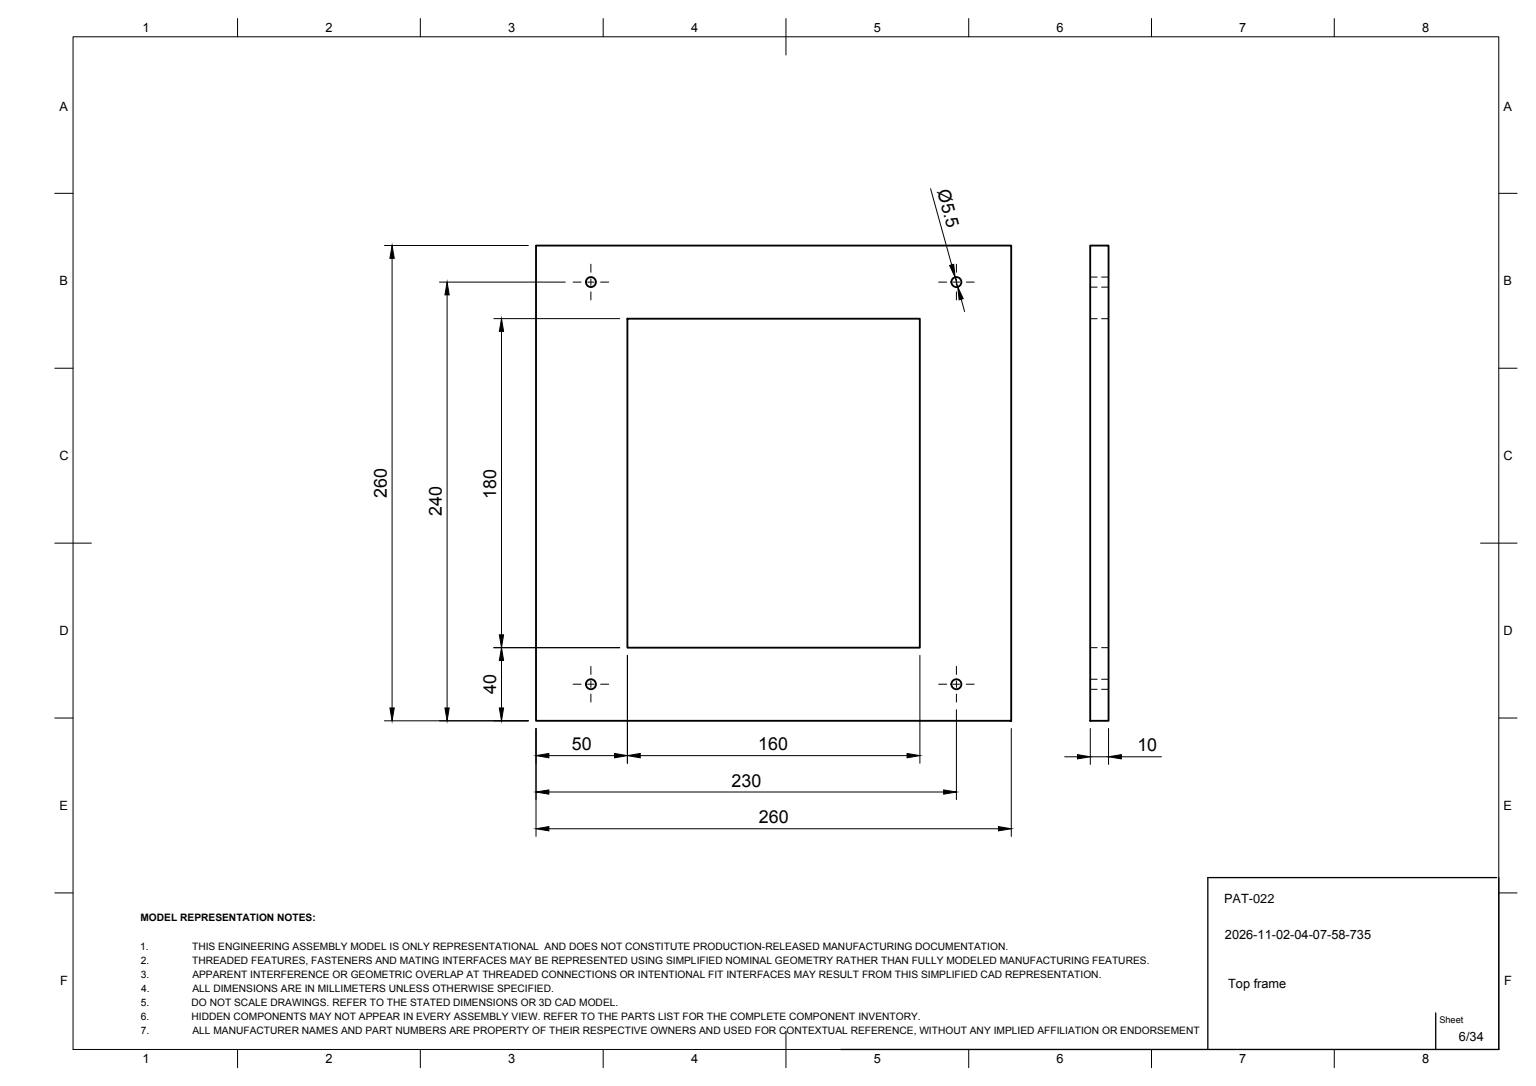
ISO-10303-21;
HEADER;
/* Generated by software containing ST-Developer
 * from STEP Tools, Inc. (www.steptools.com) 
 */

FILE_DESCRIPTION(
/* description */ ('Chute with adjustable gate'),
/* implementation_level */ '2;1');

FILE_NAME(
/* name */ 'Top frame.step',
/* time_stamp */ '2026-10-27T10:52:28-07:00',
/* author */ (''),
/* organization */ (''),
/* preprocessor_version */ 'ST-DEVELOPER v20.2',
/* originating_system */ 'Autodesk Translation Framework v15.17.0.0',
/* authorisation */ '');

FILE_SCHEMA (('AUTOMOTIVE_DESIGN { 1 0 10303 214 3 1 1 }'));
ENDSEC;

DATA;
#10=MECHANICAL_DESIGN_GEOMETRIC_PRESENTATION_REPRESENTATION('',(#415),#13094);
#351=SHAPE_REPRESENTATION_RELATIONSHIP('SRR','None',#13252,#383);
#383=ADVANCED_BREP_SHAPE_REPRESENTATION('',(#447),#13061);
#415=STYLED_ITEM('',(#13474),#447);
#447=MANIFOLD_SOLID_BREP('Body1',#7598);
#482=FACE_BOUND('',#1360,.T.);
#483=FACE_BOUND('',#1361,.T.);
#484=FACE_BOUND('',#1362,.T.);
#485=FACE_BOUND('',#1363,.T.);
#486=FACE_BOUND('',#1364,.T.);
#487=FACE_BOUND('',#1366,.T.);
#488=FACE_BOUND('',#1367,.T.);
#489=FACE_BOUND('',#1368,.T.);
#490=FACE_BOUND('',#1369,.T.);
#491=FACE_BOUND('',#1370,.T.);
#596=PLANE('',#8020);
#597=PLANE('',#8021);
#598=PLANE('',#8022);
#599=PLANE('',#8023);
#600=PLANE('',#8024);
#601=PLANE('',#8025);
#602=PLANE('',#8026);
#603=PLANE('',#8027);
#604=PLANE('',#8028);
#605=PLANE('',#8029);
#924=FACE_OUTER_BOUND('',#1347,.T.);
#925=FACE_OUTER_BOUND('',#1348,.T.);
#926=FACE_OUTER_BOUND('',#1349,.T.);
#927=FACE_OUTER_BOUND('',#1350,.T.);
#928=FACE_OUTER_BOUND('',#1351,.T.);
#929=FACE_OUTER_BOUND('',#1352,.T.);
#930=FACE_OUTER_BOUND('',#1353,.T.);
#931=FACE_OUTER_BOUND('',#1354,.T.);
#932=FACE_OUTER_BOUND('',#1355,.T.);
#933=FACE_OUTER_BOUND('',#1356,.T.);
#934=FACE_OUTER_BOUND('',#1357,.T.);
#935=FACE_OUTER_BOUND('',#1358,.T.);
#936=FACE_OUTER_BOUND('',#1359,.T.);
#937=FACE_OUTER_BOUND('',#1365,.T.);
#1347=EDGE_LOOP('',(#5234,#5235,#5236,#5237));
#1348=EDGE_LOOP('',(#5238,#5239,#5240,#5241));
#1349=EDGE_LOOP('',(#5242,#5243,#5244,#5245));
#1350=EDGE_LOOP('',(#5246,#5247,#5248,#5249));
#1351=EDGE_LOOP('',(#5250,#5251,#5252,#5253));
#1352=EDGE_LOOP('',(#5254,#5255,#5256,#5257));
#1353=EDGE_LOOP('',(#5258,#5259,#5260,#5261));
#1354=EDGE_LOOP('',(#5262,#5263,#5264,#5265));
#1355=EDGE_LOOP('',(#5266,#5267,#5268,#5269));
#1356=EDGE_LOOP('',(#5270,#5271,#5272,#5273));
#1357=EDGE_LOOP('',(#5274,#5275,#5276,#5277));
#1358=EDGE_LOOP('',(#5278,#5279,#5280,#5281));
#1359=EDGE_LOOP('',(#5282,#5283,#5284,#5285));
#1360=EDGE_LOOP('',(#5286,#5287,#5288,#5289));
#1361=EDGE_LOOP('',(#5290));
#1362=EDGE_LOOP('',(#5291));
#1363=EDGE_LOOP('',(#5292));
#1364=EDGE_LOOP('',(#5293));
#1365=EDGE_LOOP('',(#5294,#5295,#5296,#5297));
#1366=EDGE_LOOP('',(#5298,#5299,#5300,#5301));
#1367=EDGE_LOOP('',(#5302));
#1368=EDGE_LOOP('',(#5303));
#1369=EDGE_LOOP('',(#5304));
#1370=EDGE_LOOP('',(#5305));
#1876=LINE('',#10957,#2653);
#1877=LINE('',#10963,#2654);
#1878=LINE('',#10969,#2655);
#1879=LINE('',#10975,#2656);
#1880=LINE('',#10980,#2657);
#1881=LINE('',#10982,#2658);
#1882=LINE('',#10984,#2659);
#1883=LINE('',#10985,#2660);
#1884=LINE('',#10988,#2661);
#1885=LINE('',#10990,#2662);
#1886=LINE('',#10991,#2663);
#1887=LINE('',#10994,#2664);
#1888=LINE('',#10996,#2665);
#1889=LINE('',#10997,#2666);
#1890=LINE('',#10999,#2667);
#1891=LINE('',#11000,#2668);
#1892=LINE('',#11004,#2669);
#1893=LINE('',#11006,#2670);
#1894=LINE('',#11008,#2671);
#1895=LINE('',#11009,#2672);
#1896=LINE('',#11012,#2673);
#1897=LINE('',#11014,#2674);
#1898=LINE('',#11015,#2675);
#1899=LINE('',#11018,#2676);
#1900=LINE('',#11020,#2677);
#1901=LINE('',#11021,#2678);
#1902=LINE('',#11023,#2679);
#1903=LINE('',#11024,#2680);
#2653=VECTOR('',#8762,0.274999999999999);
#2654=VECTOR('',#8769,0.275);
#2655=VECTOR('',#8776,0.275);
#2656=VECTOR('',#8783,0.274999999999999);
#2657=VECTOR('',#8788,1.);
#2658=VECTOR('',#8789,1.);
#2659=VECTOR('',#8790,1.);
#2660=VECTOR('',#8791,1.);
#2661=VECTOR('',#8794,1.);
#2662=VECTOR('',#8795,1.);
#2663=VECTOR('',#8796,1.);
#2664=VECTOR('',#8799,1.);
#2665=VECTOR('',#8800,1.);
#2666=VECTOR('',#8801,1.);
#2667=VECTOR('',#8804,1.);
#2668=VECTOR('',#8805,1.);
#2669=VECTOR('',#8808,1.);
#2670=VECTOR('',#8809,1.);
#2671=VECTOR('',#8810,1.);
#2672=VECTOR('',#8811,1.);
#2673=VECTOR('',#8814,1.);
#2674=VECTOR('',#8815,1.);
#2675=VECTOR('',#8816,1.);
#2676=VECTOR('',#8819,1.);
#2677=VECTOR('',#8820,1.);
#2678=VECTOR('',#8821,1.);
#2679=VECTOR('',#8824,1.);
#2680=VECTOR('',#8825,1.);
#3422=CIRCLE('',#8009,0.274999999999999);
#3423=CIRCLE('',#8010,0.274999999999999);
#3424=CIRCLE('',#8012,0.275);
#3425=CIRCLE('',#8013,0.275);
#3426=CIRCLE('',#8015,0.275);
#3427=CIRCLE('',#8016,0.275);
#3428=CIRCLE('',#8018,0.274999999999999);
#3429=CIRCLE('',#8019,0.274999999999999);
#3609=VERTEX_POINT('',#10954);
#3610=VERTEX_POINT('',#10956);
#3611=VERTEX_POINT('',#10960);
#3612=VERTEX_POINT('',#10962);
#3613=VERTEX_POINT('',#10966);
#3614=VERTEX_POINT('',#10968);
#3615=VERTEX_POINT('',#10972);
#3616=VERTEX_POINT('',#10974);
#3617=VERTEX_POINT('',#10978);
#3618=VERTEX_POINT('',#10979);
#3619=VERTEX_POINT('',#10981);
#3620=VERTEX_POINT('',#10983);
#3621=VERTEX_POINT('',#10987);
#3622=VERTEX_POINT('',#10989);
#3623=VERTEX_POINT('',#10993);
#3624=VERTEX_POINT('',#10995);
#3625=VERTEX_POINT('',#11002);
#3626=VERTEX_POINT('',#11003);
#3627=VERTEX_POINT('',#11005);
#3628=VERTEX_POINT('',#11007);
#3629=VERTEX_POINT('',#11011);
#3630=VERTEX_POINT('',#11013);
#3631=VERTEX_POINT('',#11017);
#3632=VERTEX_POINT('',#11019);
#4250=EDGE_CURVE('',#3609,#3609,#3422,.T.);
#4251=EDGE_CURVE('',#3609,#3610,#1876,.T.);
#4252=EDGE_CURVE('',#3610,#3610,#3423,.T.);
#4253=EDGE_CURVE('',#3611,#3611,#3424,.T.);
#4254=EDGE_CURVE('',#3611,#3612,#1877,.T.);
#4255=EDGE_CURVE('',#3612,#3612,#3425,.T.);
#4256=EDGE_CURVE('',#3613,#3613,#3426,.T.);
#4257=EDGE_CURVE('',#3613,#3614,#1878,.T.);
#4258=EDGE_CURVE('',#3614,#3614,#3427,.T.);
#4259=EDGE_CURVE('',#3615,#3615,#3428,.T.);
#4260=EDGE_CURVE('',#3615,#3616,#1879,.T.);
#4261=EDGE_CURVE('',#3616,#3616,#3429,.T.);
#4262=EDGE_CURVE('',#3617,#3618,#1880,.T.);
#4263=EDGE_CURVE('',#3619,#3617,#1881,.T.);
#4264=EDGE_CURVE('',#3620,#3619,#1882,.T.);
#4265=EDGE_CURVE('',#3620,#3618,#1883,.T.);
#4266=EDGE_CURVE('',#3618,#3621,#1884,.T.);
#4267=EDGE_CURVE('',#3622,#3620,#1885,.T.);
#4268=EDGE_CURVE('',#3622,#3621,#1886,.T.);
#4269=EDGE_CURVE('',#3621,#3623,#1887,.T.);
#4270=EDGE_CURVE('',#3624,#3622,#1888,.T.);
#4271=EDGE_CURVE('',#3624,#3623,#1889,.T.);
#4272=EDGE_CURVE('',#3623,#3617,#1890,.T.);
#4273=EDGE_CURVE('',#3619,#3624,#1891,.T.);
#4274=EDGE_CURVE('',#3625,#3626,#1892,.T.);
#4275=EDGE_CURVE('',#3626,#3627,#1893,.T.);
#4276=EDGE_CURVE('',#3628,#3627,#1894,.T.);
#4277=EDGE_CURVE('',#3625,#3628,#1895,.T.);
#4278=EDGE_CURVE('',#3629,#3625,#1896,.T.);
#4279=EDGE_CURVE('',#3630,#3628,#1897,.T.);
#4280=EDGE_CURVE('',#3629,#3630,#1898,.T.);
#4281=EDGE_CURVE('',#3631,#3629,#1899,.T.);
#4282=EDGE_CURVE('',#3632,#3630,#1900,.T.);
#4283=EDGE_CURVE('',#3631,#3632,#1901,.T.);
#4284=EDGE_CURVE('',#3626,#3631,#1902,.T.);
#4285=EDGE_CURVE('',#3627,#3632,#1903,.T.);
#5234=ORIENTED_EDGE('',*,*,#4250,.F.);
#5235=ORIENTED_EDGE('',*,*,#4251,.T.);
#5236=ORIENTED_EDGE('',*,*,#4252,.F.);
#5237=ORIENTED_EDGE('',*,*,#4251,.F.);
#5238=ORIENTED_EDGE('',*,*,#4253,.F.);
#5239=ORIENTED_EDGE('',*,*,#4254,.T.);
#5240=ORIENTED_EDGE('',*,*,#4255,.F.);
#5241=ORIENTED_EDGE('',*,*,#4254,.F.);
#5242=ORIENTED_EDGE('',*,*,#4256,.F.);
#5243=ORIENTED_EDGE('',*,*,#4257,.T.);
#5244=ORIENTED_EDGE('',*,*,#4258,.F.);
#5245=ORIENTED_EDGE('',*,*,#4257,.F.);
#5246=ORIENTED_EDGE('',*,*,#4259,.F.);
#5247=ORIENTED_EDGE('',*,*,#4260,.T.);
#5248=ORIENTED_EDGE('',*,*,#4261,.F.);
#5249=ORIENTED_EDGE('',*,*,#4260,.F.);
#5250=ORIENTED_EDGE('',*,*,#4262,.F.);
#5251=ORIENTED_EDGE('',*,*,#4263,.F.);
#5252=ORIENTED_EDGE('',*,*,#4264,.F.);
#5253=ORIENTED_EDGE('',*,*,#4265,.T.);
#5254=ORIENTED_EDGE('',*,*,#4266,.F.);
#5255=ORIENTED_EDGE('',*,*,#4265,.F.);
#5256=ORIENTED_EDGE('',*,*,#4267,.F.);
#5257=ORIENTED_EDGE('',*,*,#4268,.T.);
#5258=ORIENTED_EDGE('',*,*,#4269,.F.);
#5259=ORIENTED_EDGE('',*,*,#4268,.F.);
#5260=ORIENTED_EDGE('',*,*,#4270,.F.);
#5261=ORIENTED_EDGE('',*,*,#4271,.T.);
#5262=ORIENTED_EDGE('',*,*,#4272,.F.);
#5263=ORIENTED_EDGE('',*,*,#4271,.F.);
#5264=ORIENTED_EDGE('',*,*,#4273,.F.);
#5265=ORIENTED_EDGE('',*,*,#4263,.T.);
#5266=ORIENTED_EDGE('',*,*,#4274,.T.);
#5267=ORIENTED_EDGE('',*,*,#4275,.T.);
#5268=ORIENTED_EDGE('',*,*,#4276,.F.);
#5269=ORIENTED_EDGE('',*,*,#4277,.F.);
#5270=ORIENTED_EDGE('',*,*,#4278,.T.);
#5271=ORIENTED_EDGE('',*,*,#4277,.T.);
#5272=ORIENTED_EDGE('',*,*,#4279,.F.);
#5273=ORIENTED_EDGE('',*,*,#4280,.F.);
#5274=ORIENTED_EDGE('',*,*,#4281,.T.);
#5275=ORIENTED_EDGE('',*,*,#4280,.T.);
#5276=ORIENTED_EDGE('',*,*,#4282,.F.);
#5277=ORIENTED_EDGE('',*,*,#4283,.F.);
#5278=ORIENTED_EDGE('',*,*,#4284,.T.);
#5279=ORIENTED_EDGE('',*,*,#4283,.T.);
#5280=ORIENTED_EDGE('',*,*,#4285,.F.);
#5281=ORIENTED_EDGE('',*,*,#4275,.F.);
#5282=ORIENTED_EDGE('',*,*,#4285,.T.);
#5283=ORIENTED_EDGE('',*,*,#4282,.T.);
#5284=ORIENTED_EDGE('',*,*,#4279,.T.);
#5285=ORIENTED_EDGE('',*,*,#4276,.T.);
#5286=ORIENTED_EDGE('',*,*,#4269,.T.);
#5287=ORIENTED_EDGE('',*,*,#4272,.T.);
#5288=ORIENTED_EDGE('',*,*,#4262,.T.);
#5289=ORIENTED_EDGE('',*,*,#4266,.T.);
#5290=ORIENTED_EDGE('',*,*,#4261,.T.);
#5291=ORIENTED_EDGE('',*,*,#4258,.T.);
#5292=ORIENTED_EDGE('',*,*,#4255,.T.);
#5293=ORIENTED_EDGE('',*,*,#4252,.T.);
#5294=ORIENTED_EDGE('',*,*,#4284,.F.);
#5295=ORIENTED_EDGE('',*,*,#4274,.F.);
#5296=ORIENTED_EDGE('',*,*,#4278,.F.);
#5297=ORIENTED_EDGE('',*,*,#4281,.F.);
#5298=ORIENTED_EDGE('',*,*,#4270,.T.);
#5299=ORIENTED_EDGE('',*,*,#4267,.T.);
#5300=ORIENTED_EDGE('',*,*,#4264,.T.);
#5301=ORIENTED_EDGE('',*,*,#4273,.T.);
#5302=ORIENTED_EDGE('',*,*,#4259,.T.);
#5303=ORIENTED_EDGE('',*,*,#4256,.T.);
#5304=ORIENTED_EDGE('',*,*,#4253,.T.);
#5305=ORIENTED_EDGE('',*,*,#4250,.T.);
#7110=CYLINDRICAL_SURFACE('',#8008,0.274999999999999);
#7111=CYLINDRICAL_SURFACE('',#8011,0.275);
#7112=CYLINDRICAL_SURFACE('',#8014,0.275);
#7113=CYLINDRICAL_SURFACE('',#8017,0.274999999999999);
#7192=ADVANCED_FACE('',(#924),#7110,.F.);
#7193=ADVANCED_FACE('',(#925),#7111,.F.);
#7194=ADVANCED_FACE('',(#926),#7112,.F.);
#7195=ADVANCED_FACE('',(#927),#7113,.F.);
#7196=ADVANCED_FACE('',(#928),#596,.F.);
#7197=ADVANCED_FACE('',(#929),#597,.F.);
#7198=ADVANCED_FACE('',(#930),#598,.F.);
#7199=ADVANCED_FACE('',(#931),#599,.F.);
#7200=ADVANCED_FACE('',(#932),#600,.T.);
#7201=ADVANCED_FACE('',(#933),#601,.T.);
#7202=ADVANCED_FACE('',(#934),#602,.T.);
#7203=ADVANCED_FACE('',(#935),#603,.T.);
#7204=ADVANCED_FACE('',(#936,#482,#483,#484,#485,#486),#604,.T.);
#7205=ADVANCED_FACE('',(#937,#487,#488,#489,#490,#491),#605,.F.);
#7598=CLOSED_SHELL('',(#7192,#7193,#7194,#7195,#7196,#7197,#7198,#7199,
#7200,#7201,#7202,#7203,#7204,#7205));
#8007=AXIS2_PLACEMENT_3D('',#10952,#8756,#8757);
#8008=AXIS2_PLACEMENT_3D('',#10953,#8758,#8759);
#8009=AXIS2_PLACEMENT_3D('',#10955,#8760,#8761);
#8010=AXIS2_PLACEMENT_3D('',#10958,#8763,#8764);
#8011=AXIS2_PLACEMENT_3D('',#10959,#8765,#8766);
#8012=AXIS2_PLACEMENT_3D('',#10961,#8767,#8768);
#8013=AXIS2_PLACEMENT_3D('',#10964,#8770,#8771);
#8014=AXIS2_PLACEMENT_3D('',#10965,#8772,#8773);
#8015=AXIS2_PLACEMENT_3D('',#10967,#8774,#8775);
#8016=AXIS2_PLACEMENT_3D('',#10970,#8777,#8778);
#8017=AXIS2_PLACEMENT_3D('',#10971,#8779,#8780);
#8018=AXIS2_PLACEMENT_3D('',#10973,#8781,#8782);
#8019=AXIS2_PLACEMENT_3D('',#10976,#8784,#8785);
#8020=AXIS2_PLACEMENT_3D('',#10977,#8786,#8787);
#8021=AXIS2_PLACEMENT_3D('',#10986,#8792,#8793);
#8022=AXIS2_PLACEMENT_3D('',#10992,#8797,#8798);
#8023=AXIS2_PLACEMENT_3D('',#10998,#8802,#8803);
#8024=AXIS2_PLACEMENT_3D('',#11001,#8806,#8807);
#8025=AXIS2_PLACEMENT_3D('',#11010,#8812,#8813);
#8026=AXIS2_PLACEMENT_3D('',#11016,#8817,#8818);
#8027=AXIS2_PLACEMENT_3D('',#11022,#8822,#8823);
#8028=AXIS2_PLACEMENT_3D('',#11025,#8826,#8827);
#8029=AXIS2_PLACEMENT_3D('',#11026,#8828,#8829);
#8756=DIRECTION('axis',(0.,0.,1.));
#8757=DIRECTION('refdir',(1.,0.,0.));
#8758=DIRECTION('center_axis',(0.,0.,1.));
#8759=DIRECTION('ref_axis',(1.,0.,0.));
#8760=DIRECTION('center_axis',(0.,0.,1.));
#8761=DIRECTION('ref_axis',(1.,0.,0.));
#8762=DIRECTION('',(0.,0.,1.));
#8763=DIRECTION('center_axis',(0.,0.,-1.));
#8764=DIRECTION('ref_axis',(1.,0.,0.));
#8765=DIRECTION('center_axis',(0.,0.,1.));
#8766=DIRECTION('ref_axis',(1.,0.,0.));
#8767=DIRECTION('center_axis',(0.,0.,1.));
#8768=DIRECTION('ref_axis',(1.,0.,0.));
#8769=DIRECTION('',(0.,0.,1.));
#8770=DIRECTION('center_axis',(0.,0.,-1.));
#8771=DIRECTION('ref_axis',(1.,0.,0.));
#8772=DIRECTION('center_axis',(0.,0.,1.));
#8773=DIRECTION('ref_axis',(1.,0.,0.));
#8774=DIRECTION('center_axis',(0.,0.,1.));
#8775=DIRECTION('ref_axis',(1.,0.,0.));
#8776=DIRECTION('',(0.,0.,1.));
#8777=DIRECTION('center_axis',(0.,0.,-1.));
#8778=DIRECTION('ref_axis',(1.,0.,0.));
#8779=DIRECTION('center_axis',(0.,0.,1.));
#8780=DIRECTION('ref_axis',(1.,0.,0.));
#8781=DIRECTION('center_axis',(0.,0.,1.));
#8782=DIRECTION('ref_axis',(1.,0.,0.));
#8783=DIRECTION('',(0.,0.,1.));
#8784=DIRECTION('center_axis',(0.,0.,-1.));
#8785=DIRECTION('ref_axis',(1.,0.,0.));
#8786=DIRECTION('center_axis',(0.,-1.,0.));
#8787=DIRECTION('ref_axis',(1.,0.,0.));
#8788=DIRECTION('',(-1.,0.,0.));
#8789=DIRECTION('',(0.,0.,1.));
#8790=DIRECTION('',(1.,0.,0.));
#8791=DIRECTION('',(0.,0.,1.));
#8792=DIRECTION('center_axis',(-1.,0.,0.));
#8793=DIRECTION('ref_axis',(0.,-1.,0.));
#8794=DIRECTION('',(0.,1.,0.));
#8795=DIRECTION('',(0.,-1.,0.));
#8796=DIRECTION('',(0.,0.,1.));
#8797=DIRECTION('center_axis',(0.,1.,0.));
#8798=DIRECTION('ref_axis',(-1.,0.,0.));
#8799=DIRECTION('',(1.,0.,0.));
#8800=DIRECTION('',(-1.,0.,0.));
#8801=DIRECTION('',(0.,0.,1.));
#8802=DIRECTION('center_axis',(1.,0.,0.));
#8803=DIRECTION('ref_axis',(0.,1.,0.));
#8804=DIRECTION('',(0.,-1.,0.));
#8805=DIRECTION('',(0.,1.,0.));
#8806=DIRECTION('center_axis',(0.,1.,0.));
#8807=DIRECTION('ref_axis',(-1.,0.,0.));
#8808=DIRECTION('',(-1.,0.,0.));
#8809=DIRECTION('',(0.,0.,1.));
#8810=DIRECTION('',(-1.,0.,0.));
#8811=DIRECTION('',(0.,0.,1.));
#8812=DIRECTION('center_axis',(1.,0.,0.));
#8813=DIRECTION('ref_axis',(0.,1.,0.));
#8814=DIRECTION('',(0.,1.,0.));
#8815=DIRECTION('',(0.,1.,0.));
#8816=DIRECTION('',(0.,0.,1.));
#8817=DIRECTION('center_axis',(0.,-1.,0.));
#8818=DIRECTION('ref_axis',(1.,0.,0.));
#8819=DIRECTION('',(1.,0.,0.));
#8820=DIRECTION('',(1.,0.,0.));
#8821=DIRECTION('',(0.,0.,1.));
#8822=DIRECTION('center_axis',(-1.,0.,0.));
#8823=DIRECTION('ref_axis',(0.,-1.,0.));
#8824=DIRECTION('',(0.,-1.,0.));
#8825=DIRECTION('',(0.,-1.,0.));
#8826=DIRECTION('center_axis',(0.,0.,1.));
#8827=DIRECTION('ref_axis',(1.,0.,0.));
#8828=DIRECTION('center_axis',(0.,0.,1.));
#8829=DIRECTION('ref_axis',(1.,0.,0.));
#10952=CARTESIAN_POINT('',(0.,0.,0.));
#10953=CARTESIAN_POINT('Origin',(23.,-11.,39.9));
#10954=CARTESIAN_POINT('',(22.725,-11.,40.));
#10955=CARTESIAN_POINT('Origin',(23.,-11.,40.));
#10956=CARTESIAN_POINT('',(22.725,-11.,41.));
#10957=CARTESIAN_POINT('',(22.725,-11.,39.9));
#10958=CARTESIAN_POINT('Origin',(23.,-11.,41.));
#10959=CARTESIAN_POINT('Origin',(3.,11.,39.9));
#10960=CARTESIAN_POINT('',(2.725,11.,40.));
#10961=CARTESIAN_POINT('Origin',(3.,11.,40.));
#10962=CARTESIAN_POINT('',(2.725,11.,41.));
#10963=CARTESIAN_POINT('',(2.725,11.,39.9));
#10964=CARTESIAN_POINT('Origin',(3.,11.,41.));
#10965=CARTESIAN_POINT('Origin',(3.,-11.,39.9));
#10966=CARTESIAN_POINT('',(2.725,-11.,40.));
#10967=CARTESIAN_POINT('Origin',(3.,-11.,40.));
#10968=CARTESIAN_POINT('',(2.725,-11.,41.));
#10969=CARTESIAN_POINT('',(2.725,-11.,39.9));
#10970=CARTESIAN_POINT('Origin',(3.,-11.,41.));
#10971=CARTESIAN_POINT('Origin',(23.,11.,39.9));
#10972=CARTESIAN_POINT('',(22.725,11.,40.));
#10973=CARTESIAN_POINT('Origin',(23.,11.,40.));
#10974=CARTESIAN_POINT('',(22.725,11.,41.));
#10975=CARTESIAN_POINT('',(22.725,11.,39.9));
#10976=CARTESIAN_POINT('Origin',(23.,11.,41.));
#10977=CARTESIAN_POINT('Origin',(5.,-9.,39.9));
#10978=CARTESIAN_POINT('',(21.,-9.,41.));
#10979=CARTESIAN_POINT('',(5.,-9.,41.));
#10980=CARTESIAN_POINT('',(9.,-9.,41.));
#10981=CARTESIAN_POINT('',(21.,-9.,40.));
#10982=CARTESIAN_POINT('',(21.,-9.,39.9));
#10983=CARTESIAN_POINT('',(5.,-9.,40.));
#10984=CARTESIAN_POINT('',(9.,-9.,40.));
#10985=CARTESIAN_POINT('',(5.,-9.,39.9));
#10986=CARTESIAN_POINT('Origin',(5.,9.,39.9));
#10987=CARTESIAN_POINT('',(5.,9.,41.));
#10988=CARTESIAN_POINT('',(5.,4.5,41.));
#10989=CARTESIAN_POINT('',(5.,9.,40.));
#10990=CARTESIAN_POINT('',(5.,4.5,40.));
#10991=CARTESIAN_POINT('',(5.,9.,39.9));
#10992=CARTESIAN_POINT('Origin',(21.,9.,39.9));
#10993=CARTESIAN_POINT('',(21.,9.,41.));
#10994=CARTESIAN_POINT('',(17.,9.,41.));
#10995=CARTESIAN_POINT('',(21.,9.,40.));
#10996=CARTESIAN_POINT('',(17.,9.,40.));
#10997=CARTESIAN_POINT('',(21.,9.,39.9));
#10998=CARTESIAN_POINT('Origin',(21.,-9.,39.9));
#10999=CARTESIAN_POINT('',(21.,-4.5,41.));
#11000=CARTESIAN_POINT('',(21.,-4.5,40.));
#11001=CARTESIAN_POINT('Origin',(26.,13.,40.));
#11002=CARTESIAN_POINT('',(26.,13.,40.));
#11003=CARTESIAN_POINT('',(0.,13.,40.));
#11004=CARTESIAN_POINT('',(26.,13.,40.));
#11005=CARTESIAN_POINT('',(0.,13.,41.));
#11006=CARTESIAN_POINT('',(0.,13.,40.));
#11007=CARTESIAN_POINT('',(26.,13.,41.));
#11008=CARTESIAN_POINT('',(26.,13.,41.));
#11009=CARTESIAN_POINT('',(26.,13.,40.));
#11010=CARTESIAN_POINT('Origin',(26.,-13.,40.));
#11011=CARTESIAN_POINT('',(26.,-13.,40.));
#11012=CARTESIAN_POINT('',(26.,-13.,40.));
#11013=CARTESIAN_POINT('',(26.,-13.,41.));
#11014=CARTESIAN_POINT('',(26.,-13.,41.));
#11015=CARTESIAN_POINT('',(26.,-13.,40.));
#11016=CARTESIAN_POINT('Origin',(0.,-13.,40.));
#11017=CARTESIAN_POINT('',(0.,-13.,40.));
#11018=CARTESIAN_POINT('',(0.,-13.,40.));
#11019=CARTESIAN_POINT('',(0.,-13.,41.));
#11020=CARTESIAN_POINT('',(0.,-13.,41.));
#11021=CARTESIAN_POINT('',(0.,-13.,40.));
#11022=CARTESIAN_POINT('Origin',(0.,13.,40.));
#11023=CARTESIAN_POINT('',(0.,13.,40.));
#11024=CARTESIAN_POINT('',(0.,13.,41.));
#11025=CARTESIAN_POINT('Origin',(13.,0.,41.));
#11026=CARTESIAN_POINT('Origin',(13.,0.,40.));
#13024=UNCERTAINTY_MEASURE_WITH_UNIT(LENGTH_MEASURE(0.001),#13095,
'DISTANCE_ACCURACY_VALUE',
'Maximum model space distance between geometric entities at asserted c
onnectivities');
#13057=UNCERTAINTY_MEASURE_WITH_UNIT(LENGTH_MEASURE(0.001),#13095,
'DISTANCE_ACCURACY_VALUE',
'Maximum model space distance between geometric entities at asserted c
onnectivities');
#13061=(
GEOMETRIC_REPRESENTATION_CONTEXT(3)
GLOBAL_UNCERTAINTY_ASSIGNED_CONTEXT((#13024))
GLOBAL_UNIT_ASSIGNED_CONTEXT((#13095,#13097,#13098))
REPRESENTATION_CONTEXT('','3D')
);
#13094=(
GEOMETRIC_REPRESENTATION_CONTEXT(3)
GLOBAL_UNCERTAINTY_ASSIGNED_CONTEXT((#13057))
GLOBAL_UNIT_ASSIGNED_CONTEXT((#13095,#13097,#13098))
REPRESENTATION_CONTEXT('','3D')
);
#13095=(
LENGTH_UNIT()
NAMED_UNIT(*)
SI_UNIT(.CENTI.,.METRE.)
);
#13097=(
NAMED_UNIT(*)
PLANE_ANGLE_UNIT()
SI_UNIT($,.RADIAN.)
);
#13098=(
NAMED_UNIT(*)
SI_UNIT($,.STERADIAN.)
SOLID_ANGLE_UNIT()
);
#13102=SHAPE_DEFINITION_REPRESENTATION(#13138,#13252);
#13138=PRODUCT_DEFINITION_SHAPE('',$,#13289);
#13252=SHAPE_REPRESENTATION('',(#8007),#13061);
#13285=PRODUCT_DEFINITION_CONTEXT('part definition',#13395,'design');
#13289=PRODUCT_DEFINITION('Top frame','Top frame',#13325,#13285);
#13325=PRODUCT_DEFINITION_FORMATION('',$,#13400);
#13395=APPLICATION_CONTEXT(
'Core Data for Automotive Mechanical Design Process');
#13396=PRODUCT_CONTEXT('part definition',#13395,'mechanical');
#13400=PRODUCT('Top frame','Top frame','Top frame',(#13396));
#13468=COLOUR_RGB('Dark Blue',0.08,0.2,0.34);
#13469=FILL_AREA_STYLE_COLOUR('',#13468);
#13470=FILL_AREA_STYLE('',(#13469));
#13471=SURFACE_STYLE_FILL_AREA(#13470);
#13472=SURFACE_SIDE_STYLE('',(#13471));
#13473=SURFACE_STYLE_USAGE(.BOTH.,#13472);
#13474=PRESENTATION_STYLE_ASSIGNMENT((#13473));
ENDSEC;
END-ISO-10303-21;
